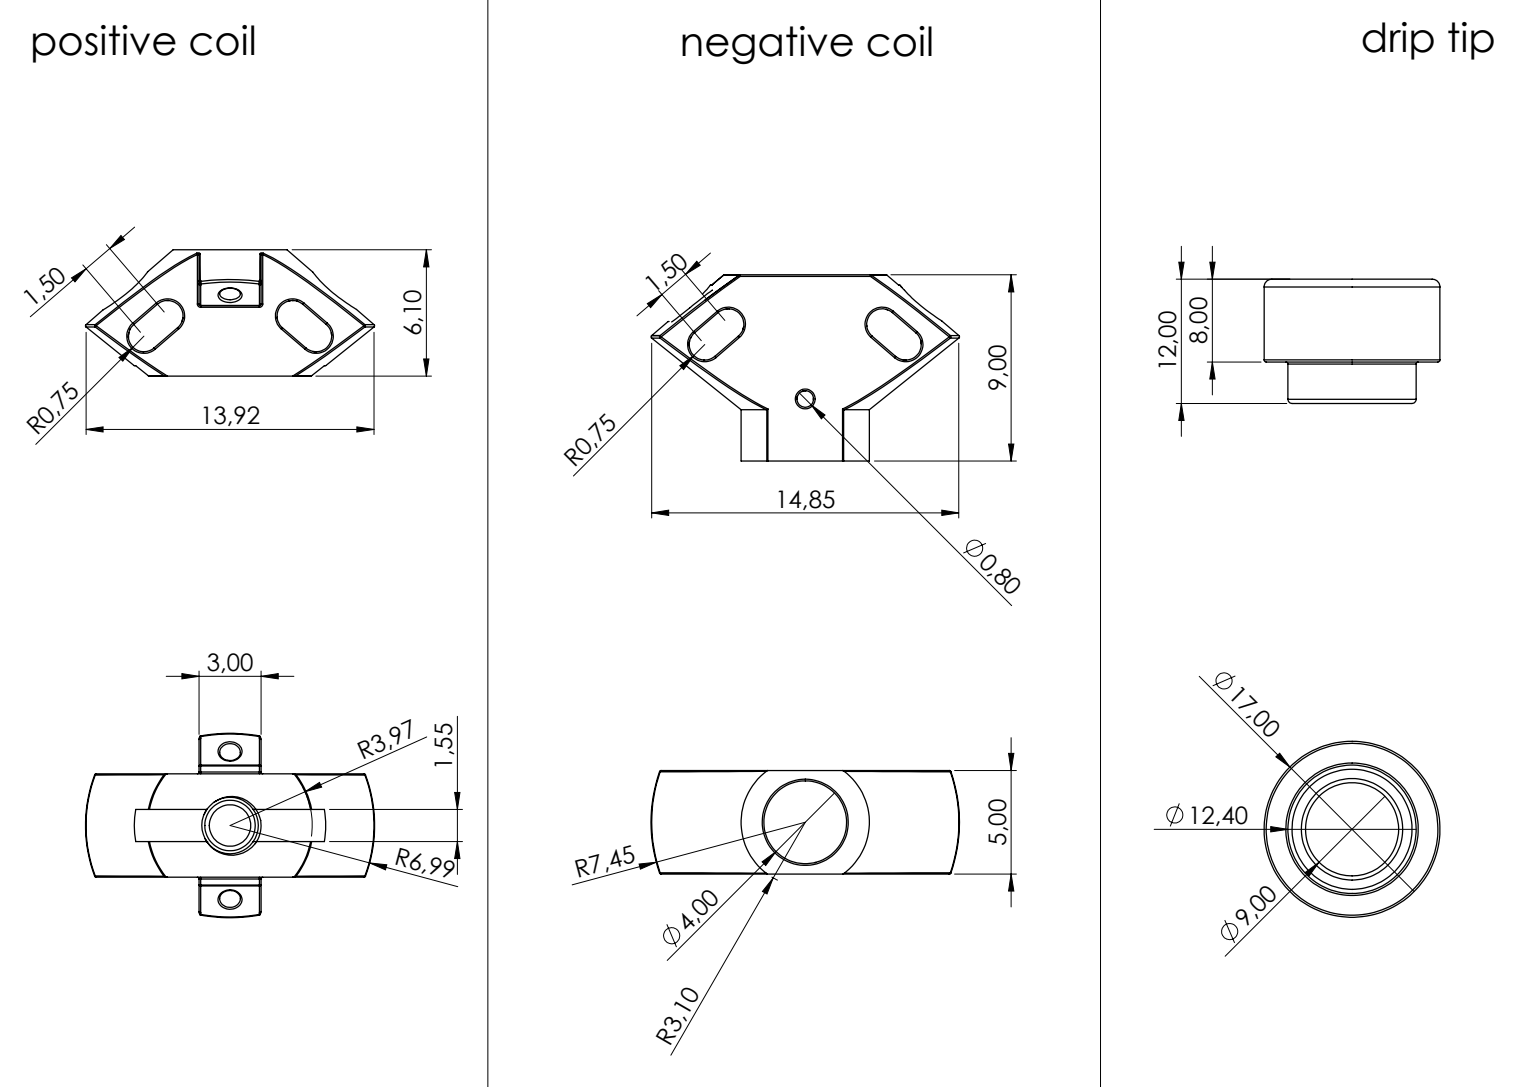
ISO-10303-21;
HEADER;
FILE_DESCRIPTION (('STEP AP214'),
    '1' );
FILE_NAME ('drip tip.step',
    '2026-10-05T20:10:51',
    ( '' ),
    ( '' ),
    'SwSTEP 2.0',
    'SolidWorks 2020',
    '' );
FILE_SCHEMA (( 'AUTOMOTIVE_DESIGN' ));
ENDSEC;

DATA;
#264=CARTESIAN_POINT ( 'NONE',  ( 0.000000000000000000, 6.999999999999992006, 4.500000000000000000 ) ) ;
#345=( NAMED_UNIT ( * ) PLANE_ANGLE_UNIT ( ) SI_UNIT ( $, .RADIAN. ) );
#574=EDGE_CURVE ( 'NONE', #72143, #200201, #108968, .T. ) ;
#1305=CARTESIAN_POINT ( 'NONE',  ( 0.000000000000000000, 10.00000000000000888, 0.000000000000000000 ) ) ;
#1373=EDGE_CURVE ( 'NONE', #149611, #126977, #18598, .T. ) ;
#1519=CARTESIAN_POINT ( 'NONE',  ( 0.000000000000000000, 6.999999999999992006, 0.000000000000000000 ) ) ;
#2109=VERTEX_POINT ( 'NONE', #48401 ) ;
#2320=CARTESIAN_POINT ( 'NONE',  ( 0.000000000000000000, -3.600000000000005862, 0.000000000000000000 ) ) ;
#2591=EDGE_CURVE ( 'NONE', #127623, #140029, #92727, .T. ) ;
#3387=DIRECTION ( 'NONE',  ( 0.000000000000000000, 0.000000000000000000, 1.000000000000000000 ) ) ;
#3603=ADVANCED_FACE ( 'NONE', ( #77901 ), #61609, .T. ) ;
#3770=ADVANCED_FACE ( 'NONE', ( #43300, #210018 ), #44358, .F. ) ;
#3987=CARTESIAN_POINT ( 'NONE',  ( 0.000000000000000000, 6.999999999999992006, 0.000000000000000000 ) ) ;
#4305=FACE_BOUND ( 'NONE', #212026, .T. ) ;
#4938=DIRECTION ( 'NONE',  ( 0.000000000000000000, 0.000000000000000000, 1.000000000000000000 ) ) ;
#5232=DIRECTION ( 'NONE',  ( 0.000000000000000000, -1.000000000000000000, 0.000000000000000000 ) ) ;
#5776=AXIS2_PLACEMENT_3D ( 'NONE', #186216, #103926, #18384 ) ;
#5884=( GEOMETRIC_REPRESENTATION_CONTEXT ( 3 ) GLOBAL_UNCERTAINTY_ASSIGNED_CONTEXT ( ( #116588 ) ) GLOBAL_UNIT_ASSIGNED_CONTEXT ( ( #15813, #115528, #82956 ) ) REPRESENTATION_CONTEXT ( 'NONE', 'WORKASPACE' ) );
#6450=CARTESIAN_POINT ( 'NONE',  ( 7.837739514543059934E-16, -0.2000000000000057288, -6.399999999999999467 ) ) ;
#7360=AXIS2_PLACEMENT_3D ( 'NONE', #71860, #19921, #90286 ) ;
#7540=ADVANCED_FACE ( 'NONE', ( #18411 ), #133280, .F. ) ;
#7671=CARTESIAN_POINT ( 'NONE',  ( 0.000000000000000000, 6.999999999999992006, 0.000000000000000000 ) ) ;
#7758=VECTOR ( 'NONE', #72110, 1000.000000000000000 ) ;
#8001=VECTOR ( 'NONE', #60877, 1000.000000000000000 ) ;
#8061=CIRCLE ( 'NONE', #129250, 7.750000000000000888 ) ;
#8134=VERTEX_POINT ( 'NONE', #207931 ) ;
#8319=CARTESIAN_POINT ( 'NONE',  ( 0.000000000000000000, -2.859583229930517945E-15, 6.399999999999999467 ) ) ;
#8641=AXIS2_PLACEMENT_3D ( 'NONE', #31169, #131895, #29033 ) ;
#9557=EDGE_LOOP ( 'NONE', ( #101500, #18562 ) ) ;
#9612=DIRECTION ( 'NONE',  ( 0.000000000000000000, 0.000000000000000000, 1.000000000000000000 ) ) ;
#9696=DIRECTION ( 'NONE',  ( 0.000000000000000000, 0.000000000000000000, 1.000000000000000000 ) ) ;
#9815=FACE_OUTER_BOUND ( 'NONE', #133822, .T. ) ;
#9854=DIRECTION ( 'NONE',  ( 0.000000000000000000, 0.000000000000000000, -1.000000000000000000 ) ) ;
#10274=EDGE_CURVE ( 'NONE', #26370, #93781, #171269, .T. ) ;
#10560=ORIENTED_EDGE ( 'NONE', *, *, #10274, .F. ) ;
#10650=ORIENTED_EDGE ( 'NONE', *, *, #170575, .T. ) ;
#10651=AXIS2_PLACEMENT_3D ( 'NONE', #60312, #126471, #44089 ) ;
#11410=EDGE_CURVE ( 'NONE', #127623, #2109, #69198, .T. ) ;
#11539=CIRCLE ( 'NONE', #136023, 0.4000000000000001887 ) ;
#11722=DIRECTION ( 'NONE',  ( 0.000000000000000000, -1.000000000000000000, 0.000000000000000000 ) ) ;
#12006=EDGE_CURVE ( 'NONE', #164855, #93781, #55325, .T. ) ;
#13222=CYLINDRICAL_SURFACE ( 'NONE', #176127, 8.500000000000000000 ) ;
#13360=DIRECTION ( 'NONE',  ( 0.000000000000000000, 0.000000000000000000, -1.000000000000000000 ) ) ;
#13864=DIRECTION ( 'NONE',  ( 0.000000000000000000, 0.000000000000000000, 1.000000000000000000 ) ) ;
#14011=CARTESIAN_POINT ( 'NONE',  ( 0.000000000000000000, 7.999999999999992895, 0.000000000000000000 ) ) ;
#14188=CIRCLE ( 'NONE', #135302, 0.4000000000000001887 ) ;
#14192=DIRECTION ( 'NONE',  ( 1.000000000000000000, -0.000000000000000000, 1.224646799147353207E-16 ) ) ;
#14250=CARTESIAN_POINT ( 'NONE',  ( 0.000000000000000000, -4.000000000000003553, 0.000000000000000000 ) ) ;
#15020=CARTESIAN_POINT ( 'NONE',  ( 1.028703311283776586E-15, 0.000000000000000000, -8.300000000000000711 ) ) ;
#15073=EDGE_CURVE ( 'NONE', #23490, #200201, #150501, .T. ) ;
#15171=AXIS2_PLACEMENT_3D ( 'NONE', #14250, #80343, #32656 ) ;
#15196=DIRECTION ( 'NONE',  ( 0.000000000000000000, 0.000000000000000000, 1.000000000000000000 ) ) ;
#15813=( LENGTH_UNIT ( ) NAMED_UNIT ( * ) SI_UNIT ( .MILLI., .METRE. ) );
#16136=AXIS2_PLACEMENT_3D ( 'NONE', #83388, #118101, #149472 ) ;
#16497=CARTESIAN_POINT ( 'NONE',  ( 7.592810154713589835E-16, -0.2000000000000057288, -6.200000000000000178 ) ) ;
#16828=EDGE_CURVE ( 'NONE', #71815, #212637, #195967, .T. ) ;
#16875=PRESENTATION_STYLE_ASSIGNMENT (( #180474 ) ) ;
#16964=ORIENTED_EDGE ( 'NONE', *, *, #574, .T. ) ;
#17327=EDGE_LOOP ( 'NONE', ( #66567, #70195, #176527, #91238 ) ) ;
#17374=DIRECTION ( 'NONE',  ( 0.000000000000000000, 0.000000000000000000, 1.000000000000000000 ) ) ;
#17603=AXIS2_PLACEMENT_3D ( 'NONE', #196348, #163856, #51161 ) ;
#17738=AXIS2_PLACEMENT_3D ( 'NONE', #106614, #187797, #189939 ) ;
#18384=DIRECTION ( 'NONE',  ( 0.000000000000000000, 0.000000000000000000, -1.000000000000000000 ) ) ;
#18411=FACE_OUTER_BOUND ( 'NONE', #115151, .T. ) ;
#18447=DIRECTION ( 'NONE',  ( 0.000000000000000000, 1.000000000000000000, 0.000000000000000000 ) ) ;
#18562=ORIENTED_EDGE ( 'NONE', *, *, #16828, .T. ) ;
#18598=CIRCLE ( 'NONE', #188047, 8.500000000000000000 ) ;
#18751=( NAMED_UNIT ( * ) SI_UNIT ( $, .STERADIAN. ) SOLID_ANGLE_UNIT ( ) );
#18967=AXIS2_PLACEMENT_3D ( 'NONE', #44218, #41025, #107134 ) ;
#19216=MANIFOLD_SOLID_BREP ( 'Fillet3', #122762 ) ;
#19595=ORIENTED_EDGE ( 'NONE', *, *, #112110, .T. ) ;
#19921=DIRECTION ( 'NONE',  ( 0.000000000000000000, 1.000000000000000000, 0.000000000000000000 ) ) ;
#19971=CARTESIAN_POINT ( 'NONE',  ( 0.000000000000000000, 7.999999999999992895, 0.000000000000000000 ) ) ;
#20632=DIRECTION ( 'NONE',  ( 0.000000000000000000, 1.000000000000000000, 0.000000000000000000 ) ) ;
#20648=VERTEX_POINT ( 'NONE', #121412 ) ;
#21650=DIRECTION ( 'NONE',  ( 0.000000000000000000, 0.000000000000000000, 1.000000000000000000 ) ) ;
#22091=ORIENTED_EDGE ( 'NONE', *, *, #182300, .F. ) ;
#22316=ORIENTED_EDGE ( 'NONE', *, *, #129911, .F. ) ;
#22969=CARTESIAN_POINT ( 'NONE',  ( 1.040949779275250140E-15, 7.250000000000006217, 8.500000000000000000 ) ) ;
#23415=EDGE_CURVE ( 'NONE', #172991, #155330, #176228, .T. ) ;
#23490=VERTEX_POINT ( 'NONE', #203951 ) ;
#23563=DIRECTION ( 'NONE',  ( 0.000000000000000000, 1.000000000000000000, 0.000000000000000000 ) ) ;
#24294=( GEOMETRIC_REPRESENTATION_CONTEXT ( 3 ) GLOBAL_UNCERTAINTY_ASSIGNED_CONTEXT ( ( #165204 ) ) GLOBAL_UNIT_ASSIGNED_CONTEXT ( ( #49154, #167164, #18751 ) ) REPRESENTATION_CONTEXT ( 'NONE', 'WORKASPACE' ) );
#24424=EDGE_CURVE ( 'NONE', #186457, #26370, #72606, .T. ) ;
#25000=AXIS2_PLACEMENT_3D ( 'NONE', #1305, #30653, #194198 ) ;
#25013=CARTESIAN_POINT ( 'NONE',  ( 0.000000000000000000, -4.000000000000003553, 6.200000000000000178 ) ) ;
#25180=CIRCLE ( 'NONE', #153201, 4.500000000000000000 ) ;
#25539=AXIS2_PLACEMENT_3D ( 'NONE', #92231, #106371, #172394 ) ;
#25943=FACE_OUTER_BOUND ( 'NONE', #203281, .T. ) ;
#26067=AXIS2_PLACEMENT_3D ( 'NONE', #122402, #89831, #9612 ) ;
#26099=ORIENTED_EDGE ( 'NONE', *, *, #129911, .T. ) ;
#26104=EDGE_LOOP ( 'NONE', ( #106132, #155824 ) ) ;
#26370=VERTEX_POINT ( 'NONE', #72434 ) ;
#27243=EDGE_LOOP ( 'NONE', ( #151851, #145363, #68319, #56562 ) ) ;
#27318=ORIENTED_EDGE ( 'NONE', *, *, #175406, .F. ) ;
#28088=ADVANCED_FACE ( 'NONE', ( #103376 ), #151075, .T. ) ;
#28593=VECTOR ( 'NONE', #183309, 1000.000000000000114 ) ;
#28786=ORIENTED_EDGE ( 'NONE', *, *, #197101, .F. ) ;
#29033=DIRECTION ( 'NONE',  ( 0.000000000000000000, 0.000000000000000000, 1.000000000000000000 ) ) ;
#29391=DIRECTION ( 'NONE',  ( 0.000000000000000000, 0.000000000000000000, -1.000000000000000000 ) ) ;
#29487=FACE_OUTER_BOUND ( 'NONE', #59958, .T. ) ;
#29491=ORIENTED_EDGE ( 'NONE', *, *, #2591, .F. ) ;
#29764=EDGE_LOOP ( 'NONE', ( #129103, #156266, #53842, #117131 ) ) ;
#30232=DIRECTION ( 'NONE',  ( 0.000000000000000000, 1.000000000000000000, 0.000000000000000000 ) ) ;
#30647=DIRECTION ( 'NONE',  ( 0.000000000000000000, 1.000000000000000000, 0.000000000000000000 ) ) ;
#30653=DIRECTION ( 'NONE',  ( 0.000000000000000000, -1.000000000000000000, 0.000000000000000000 ) ) ;
#30738=CARTESIAN_POINT ( 'NONE',  ( 0.000000000000000000, -4.000000000000005329, -4.899999999999999467 ) ) ;
#31169=CARTESIAN_POINT ( 'NONE',  ( 0.000000000000000000, 6.999999999999992006, 0.000000000000000000 ) ) ;
#31690=PRODUCT ( 'drip tip', 'drip tip', '', ( #82954 ) ) ;
#31977=CARTESIAN_POINT ( 'NONE',  ( 7.102951435054647665E-16, -3.600000000000005862, 5.799999999999999822 ) ) ;
#32090=EDGE_CURVE ( 'NONE', #20648, #185214, #46033, .T. ) ;
#32238=AXIS2_PLACEMENT_3D ( 'NONE', #93763, #127396, #73202 ) ;
#32423=DIRECTION ( 'NONE',  ( 0.000000000000000000, 0.000000000000000000, 1.000000000000000000 ) ) ;
#32656=DIRECTION ( 'NONE',  ( 0.000000000000000000, 0.000000000000000000, -1.000000000000000000 ) ) ;
#32807=DIRECTION ( 'NONE',  ( 0.000000000000000000, 0.000000000000000000, -1.000000000000000000 ) ) ;
#33263=EDGE_LOOP ( 'NONE', ( #160788, #202164 ) ) ;
#33961=DIRECTION ( 'NONE',  ( 0.000000000000000000, -1.000000000000000000, 0.000000000000000000 ) ) ;
#34059=DIRECTION ( 'NONE',  ( 0.000000000000000000, -1.000000000000000000, 0.000000000000000000 ) ) ;
#34206=SURFACE_STYLE_FILL_AREA ( #64591 ) ;
#34411=AXIS2_PLACEMENT_3D ( 'NONE', #199703, #200761, #52411 ) ;
#34430=VECTOR ( 'NONE', #188585, 1000.000000000000000 ) ;
#34590=DIRECTION ( 'NONE',  ( 8.659560562354940254E-17, 0.7071067811865469066, -0.7071067811865481278 ) ) ;
#36222=DIRECTION ( 'NONE',  ( 0.000000000000000000, -1.000000000000000000, 0.000000000000000000 ) ) ;
#36564=DIRECTION ( 'NONE',  ( 1.000000000000000000, 0.000000000000000000, -1.224646799147353207E-16 ) ) ;
#36794=DIRECTION ( 'NONE',  ( 0.000000000000000000, -1.000000000000000000, 0.000000000000000000 ) ) ;
#36987=ORIENTED_EDGE ( 'NONE', *, *, #40952, .T. ) ;
#37772=CARTESIAN_POINT ( 'NONE',  ( 0.000000000000000000, 10.00000000000000888, -4.500000000000000000 ) ) ;
#38119=CARTESIAN_POINT ( 'NONE',  ( 7.592810154713589835E-16, -3.600000000000005862, -6.200000000000000178 ) ) ;
#38330=CARTESIAN_POINT ( 'NONE',  ( 0.000000000000000000, -3.600000000000005862, 0.000000000000000000 ) ) ;
#39003=CIRCLE ( 'NONE', #70207, 0.1999999999999996503 ) ;
#39310=ORIENTED_EDGE ( 'NONE', *, *, #12006, .F. ) ;
#39390=FACE_OUTER_BOUND ( 'NONE', #145990, .T. ) ;
#39682=CIRCLE ( 'NONE', #74325, 8.500000000000000000 ) ;
#39879=CARTESIAN_POINT ( 'NONE',  ( 7.837739514543059934E-16, -2.859583229930517945E-15, -6.399999999999999467 ) ) ;
#40809=TOROIDAL_SURFACE ( 'NONE', #193078, 4.899999999999999467, 0.4000000000000000222 ) ;
#40952=EDGE_CURVE ( 'NONE', #93781, #164855, #200207, .T. ) ;
#41025=DIRECTION ( 'NONE',  ( -0.000000000000000000, 1.000000000000000000, -0.000000000000000000 ) ) ;
#41110=DIRECTION ( 'NONE',  ( -1.000000000000000000, -0.000000000000000000, -0.000000000000000000 ) ) ;
#41149=AXIS2_PLACEMENT_3D ( 'NONE', #200524, #52170, #3387 ) ;
#41923=DIRECTION ( 'NONE',  ( 0.000000000000000000, 0.000000000000000000, 1.000000000000000000 ) ) ;
#42907=ADVANCED_FACE ( 'NONE', ( #29487 ), #13222, .T. ) ;
#42957=TOROIDAL_SURFACE ( 'NONE', #63644, 8.300000000000000711, 0.2000000000000000111 ) ;
#43300=FACE_BOUND ( 'NONE', #9557, .T. ) ;
#43703=DIRECTION ( 'NONE',  ( 0.000000000000000000, 0.000000000000000000, 1.000000000000000000 ) ) ;
#44089=DIRECTION ( 'NONE',  ( 0.000000000000000000, 0.000000000000000000, 1.000000000000000000 ) ) ;
#44218=CARTESIAN_POINT ( 'NONE',  ( 0.000000000000000000, -4.000000000000003553, 0.000000000000000000 ) ) ;
#44358=PLANE ( 'NONE',  #151465 ) ;
#44912=ORIENTED_EDGE ( 'NONE', *, *, #191183, .F. ) ;
#45289=DIRECTION ( 'NONE',  ( 1.224646799147353454E-16, 0.000000000000000000, -1.000000000000000000 ) ) ;
#45646=ORIENTED_EDGE ( 'NONE', *, *, #24424, .F. ) ;
#45992=AXIS2_PLACEMENT_3D ( 'NONE', #166851, #18447, #136493 ) ;
#45996=AXIS2_PLACEMENT_3D ( 'NONE', #1519, #82797, #197608 ) ;
#46033=CIRCLE ( 'NONE', #32238, 4.500000000000000000 ) ;
#46107=DIRECTION ( 'NONE',  ( 1.000000000000000000, 0.000000000000000000, -1.224646799147353207E-16 ) ) ;
#46353=DIRECTION ( 'NONE',  ( 1.000000000000000000, -0.000000000000000000, 1.224646799147353207E-16 ) ) ;
#46679=ORIENTED_EDGE ( 'NONE', *, *, #40952, .F. ) ;
#47576=AXIS2_PLACEMENT_3D ( 'NONE', #3987, #182755, #200066 ) ;
#48401=CARTESIAN_POINT ( 'NONE',  ( 9.950255243072246565E-16, 7.999999999999992895, -7.750000000000000888 ) ) ;
#48862=CARTESIAN_POINT ( 'NONE',  ( 1.016456843292303031E-15, 0.2000000000000057288, -8.300000000000000711 ) ) ;
#49154=( LENGTH_UNIT ( ) NAMED_UNIT ( * ) SI_UNIT ( .MILLI., .METRE. ) );
#50211=( NAMED_UNIT ( * ) SI_UNIT ( $, .STERADIAN. ) SOLID_ANGLE_UNIT ( ) );
#51161=DIRECTION ( 'NONE',  ( 0.000000000000000000, 0.000000000000000000, 1.000000000000000000 ) ) ;
#51278=DIRECTION ( 'NONE',  ( -1.000000000000000000, 0.000000000000000000, 0.000000000000000000 ) ) ;
#52170=DIRECTION ( 'NONE',  ( -0.000000000000000000, -1.000000000000000000, -0.000000000000000000 ) ) ;
#52411=DIRECTION ( 'NONE',  ( 0.000000000000000000, 0.000000000000000000, -1.000000000000000000 ) ) ;
#52834=ADVANCED_FACE ( 'NONE', ( #132656 ), #177396, .F. ) ;
#53318=LINE ( 'NONE', #264, #28593 ) ;
#53399=FILL_AREA_STYLE_COLOUR ( '', #190373 ) ;
#53512=DIRECTION ( 'NONE',  ( 0.000000000000000000, 0.000000000000000000, -1.000000000000000000 ) ) ;
#53589=CIRCLE ( 'NONE', #188407, 8.500000000000000000 ) ;
#53842=ORIENTED_EDGE ( 'NONE', *, *, #175406, .T. ) ;
#55192=ADVANCED_BREP_SHAPE_REPRESENTATION ( '', ( #19216, #200407 ), #152191 ) ;
#55325=CIRCLE ( 'NONE', #131441, 6.200000000000000178 ) ;
#55431=FACE_OUTER_BOUND ( 'NONE', #211433, .T. ) ;
#55551=EDGE_CURVE ( 'NONE', #132973, #2109, #8061, .T. ) ;
#56102=CARTESIAN_POINT ( 'NONE',  ( 0.000000000000000000, 0.000000000000000000, 0.000000000000000000 ) ) ;
#56254=ORIENTED_EDGE ( 'NONE', *, *, #80870, .F. ) ;
#56298=DIRECTION ( 'NONE',  ( 1.224646799147353454E-16, 0.000000000000000000, -1.000000000000000000 ) ) ;
#56425=AXIS2_PLACEMENT_3D ( 'NONE', #78190, #94472, #162661 ) ;
#56562=ORIENTED_EDGE ( 'NONE', *, *, #57451, .F. ) ;
#56611=DIRECTION ( 'NONE',  ( -1.000000000000000000, -0.000000000000000000, -0.000000000000000000 ) ) ;
#57451=EDGE_CURVE ( 'NONE', #23490, #185214, #106026, .T. ) ;
#57610=CONICAL_SURFACE ( 'NONE', #199358, 4.500000000000000000, 0.7853981633974491672 ) ;
#58396=ORIENTED_EDGE ( 'NONE', *, *, #55551, .F. ) ;
#59841=DIRECTION ( 'NONE',  ( 0.000000000000000000, 0.000000000000000000, -1.000000000000000000 ) ) ;
#59958=EDGE_LOOP ( 'NONE', ( #175177, #175570, #88728, #105076 ) ) ;
#60312=CARTESIAN_POINT ( 'NONE',  ( 0.000000000000000000, 0.2000000000000057288, 8.300000000000000711 ) ) ;
#60877=DIRECTION ( 'NONE',  ( 0.000000000000000000, -1.000000000000000000, 0.000000000000000000 ) ) ;
#61609=TOROIDAL_SURFACE ( 'NONE', #134169, 7.750000000000000888, 0.7500000000000000000 ) ;
#62655=VECTOR ( 'NONE', #5232, 1000.000000000000000 ) ;
#62703=EDGE_LOOP ( 'NONE', ( #56254, #70105, #185472, #36987 ) ) ;
#63508=CIRCLE ( 'NONE', #87776, 0.4000000000000001887 ) ;
#63620=EDGE_CURVE ( 'NONE', #163746, #20648, #205318, .T. ) ;
#63644=AXIS2_PLACEMENT_3D ( 'NONE', #188449, #92050, #9696 ) ;
#64591=FILL_AREA_STYLE ('',( #98177 ) ) ;
#65210=ADVANCED_FACE ( 'NONE', ( #185205, #4305 ), #200386, .T. ) ;
#65319=EDGE_CURVE ( 'NONE', #71815, #164855, #39003, .T. ) ;
#65544=UNCERTAINTY_MEASURE_WITH_UNIT (LENGTH_MEASURE( 1.000000000000000082E-05 ), #116330, 'distance_accuracy_value', 'NONE');
#66252=FACE_OUTER_BOUND ( 'NONE', #17327, .T. ) ;
#66418=SURFACE_STYLE_FILL_AREA ( #199633 ) ;
#66567=ORIENTED_EDGE ( 'NONE', *, *, #112110, .F. ) ;
#67883=ORIENTED_EDGE ( 'NONE', *, *, #12006, .T. ) ;
#68319=ORIENTED_EDGE ( 'NONE', *, *, #32090, .T. ) ;
#68577=ADVANCED_FACE ( 'NONE', ( #135841 ), #181091, .T. ) ;
#69198=CIRCLE ( 'NONE', #103721, 0.7499999999999997780 ) ;
#69352=CARTESIAN_POINT ( 'NONE',  ( 0.000000000000000000, 7.250000000000006217, -8.500000000000000000 ) ) ;
#69541=CARTESIAN_POINT ( 'NONE',  ( 0.000000000000000000, -3.600000000000005862, 0.000000000000000000 ) ) ;
#69625=ADVANCED_FACE ( 'NONE', ( #55431 ), #174308, .T. ) ;
#69627=SHAPE_REPRESENTATION_RELATIONSHIP ( 'NONE' , 'NONE' ,  #188305, #55192 ) ;
#69891=ADVANCED_FACE ( 'NONE', ( #96624, #127054 ), #178931, .T. ) ;
#70105=ORIENTED_EDGE ( 'NONE', *, *, #24424, .T. ) ;
#70195=ORIENTED_EDGE ( 'NONE', *, *, #162297, .F. ) ;
#70207=AXIS2_PLACEMENT_3D ( 'NONE', #6450, #175392, #56298 ) ;
#70299=CIRCLE ( 'NONE', #56425, 8.300000000000000711 ) ;
#70727=TOROIDAL_SURFACE ( 'NONE', #191810, 4.899999999999999467, 0.4000000000000000222 ) ;
#71617=STYLED_ITEM ( 'NONE', ( #16875 ), #19216 ) ;
#71769=ORIENTED_EDGE ( 'NONE', *, *, #57451, .T. ) ;
#71815=VERTEX_POINT ( 'NONE', #39879 ) ;
#71860=CARTESIAN_POINT ( 'NONE',  ( 0.000000000000000000, 7.250000000000006217, 0.000000000000000000 ) ) ;
#72110=DIRECTION ( 'NONE',  ( 0.000000000000000000, -1.000000000000000000, 0.000000000000000000 ) ) ;
#72143=VERTEX_POINT ( 'NONE', #91850 ) ;
#72434=CARTESIAN_POINT ( 'NONE',  ( 0.000000000000000000, -3.600000000000005862, 6.200000000000000178 ) ) ;
#72606=CIRCLE ( 'NONE', #34411, 6.200000000000000178 ) ;
#72771=ADVANCED_FACE ( 'NONE', ( #123894 ), #194160, .F. ) ;
#72991=ORIENTED_EDGE ( 'NONE', *, *, #170575, .F. ) ;
#73202=DIRECTION ( 'NONE',  ( 0.000000000000000000, 0.000000000000000000, -1.000000000000000000 ) ) ;
#73702=VECTOR ( 'NONE', #23563, 1000.000000000000000 ) ;
#74162=ADVANCED_FACE ( 'NONE', ( #39390 ), #166470, .T. ) ;
#74325=AXIS2_PLACEMENT_3D ( 'NONE', #98338, #182770, #13864 ) ;
#75338=CARTESIAN_POINT ( 'NONE',  ( 5.510910596163088569E-16, 10.00000000000000888, 4.500000000000000000 ) ) ;
#76218=CARTESIAN_POINT ( 'NONE',  ( 7.347880794884118750E-16, -4.000000000000003553, 5.799999999999999822 ) ) ;
#77901=FACE_OUTER_BOUND ( 'NONE', #29764, .T. ) ;
#78190=CARTESIAN_POINT ( 'NONE',  ( 0.000000000000000000, 0.000000000000000000, 0.000000000000000000 ) ) ;
#78964=DIRECTION ( 'NONE',  ( 0.000000000000000000, 0.000000000000000000, 1.000000000000000000 ) ) ;
#79154=EDGE_LOOP ( 'NONE', ( #209645, #149612, #67883, #10560 ) ) ;
#79158=ORIENTED_EDGE ( 'NONE', *, *, #87756, .F. ) ;
#79202=ORIENTED_EDGE ( 'NONE', *, *, #163561, .F. ) ;
#79679=STYLED_ITEM ( 'NONE', ( #151982 ), #55192 ) ;
#80179=ORIENTED_EDGE ( 'NONE', *, *, #179626, .T. ) ;
#80292=VERTEX_POINT ( 'NONE', #15020 ) ;
#80343=DIRECTION ( 'NONE',  ( 0.000000000000000000, -1.000000000000000000, 0.000000000000000000 ) ) ;
#80524=CIRCLE ( 'NONE', #198166, 5.500000000000005329 ) ;
#80870=EDGE_CURVE ( 'NONE', #186457, #164855, #190333, .T. ) ;
#81525=FACE_OUTER_BOUND ( 'NONE', #79154, .T. ) ;
#82404=CARTESIAN_POINT ( 'NONE',  ( 0.000000000000000000, 0.000000000000000000, 8.300000000000000711 ) ) ;
#82529=DIRECTION ( 'NONE',  ( 0.000000000000000000, -1.000000000000000000, 0.000000000000000000 ) ) ;
#82575=FACE_OUTER_BOUND ( 'NONE', #27243, .T. ) ;
#82609=DIRECTION ( 'NONE',  ( 0.000000000000000000, -1.000000000000000000, 0.000000000000000000 ) ) ;
#82797=DIRECTION ( 'NONE',  ( 0.000000000000000000, 1.000000000000000000, 0.000000000000000000 ) ) ;
#82954=PRODUCT_CONTEXT ( 'NONE', #201209, 'mechanical' ) ;
#82956=( NAMED_UNIT ( * ) SI_UNIT ( $, .STERADIAN. ) SOLID_ANGLE_UNIT ( ) );
#83331=CARTESIAN_POINT ( 'NONE',  ( 5.510910596163088569E-16, 6.999999999999992006, -4.500000000000000000 ) ) ;
#83388=CARTESIAN_POINT ( 'NONE',  ( 0.000000000000000000, 0.000000000000000000, 0.000000000000000000 ) ) ;
#83645=EDGE_LOOP ( 'NONE', ( #177931, #80179 ) ) ;
#83982=VERTEX_POINT ( 'NONE', #30738 ) ;
#86161=SHAPE_DEFINITION_REPRESENTATION ( #128549, #188305 ) ;
#86301=CARTESIAN_POINT ( 'NONE',  ( 6.735557395310444981E-16, 7.999999999999992895, -5.500000000000002665 ) ) ;
#86971=CARTESIAN_POINT ( 'NONE',  ( 0.000000000000000000, -0.2000000000000057288, 6.399999999999999467 ) ) ;
#87756=EDGE_CURVE ( 'NONE', #23490, #163746, #150598, .T. ) ;
#87776=AXIS2_PLACEMENT_3D ( 'NONE', #108622, #56611, #122775 ) ;
#88728=ORIENTED_EDGE ( 'NONE', *, *, #192353, .T. ) ;
#89166=CIRCLE ( 'NONE', #47576, 4.500000000000000000 ) ;
#89189=DIRECTION ( 'NONE',  ( 0.000000000000000000, -1.000000000000000000, 0.000000000000000000 ) ) ;
#89831=DIRECTION ( 'NONE',  ( 0.000000000000000000, 1.000000000000000000, 0.000000000000000000 ) ) ;
#90286=DIRECTION ( 'NONE',  ( 0.000000000000000000, 0.000000000000000000, 1.000000000000000000 ) ) ;
#91238=ORIENTED_EDGE ( 'NONE', *, *, #32090, .F. ) ;
#91398=EDGE_CURVE ( 'NONE', #8134, #83982, #174578, .T. ) ;
#91569=CIRCLE ( 'NONE', #119276, 0.4000000000000001887 ) ;
#91812=CARTESIAN_POINT ( 'NONE',  ( 7.592810154713589835E-16, -4.000000000000003553, -6.200000000000000178 ) ) ;
#91850=CARTESIAN_POINT ( 'NONE',  ( 0.000000000000000000, 7.999999999999992895, 5.500000000000002665 ) ) ;
#92050=DIRECTION ( 'NONE',  ( 0.000000000000000000, 1.000000000000000000, 0.000000000000000000 ) ) ;
#92213=CARTESIAN_POINT ( 'NONE',  ( 0.000000000000000000, -3.600000000000005862, 0.000000000000000000 ) ) ;
#92231=CARTESIAN_POINT ( 'NONE',  ( 0.000000000000000000, 0.2000000000000057288, 0.000000000000000000 ) ) ;
#92573=AXIS2_PLACEMENT_3D ( 'NONE', #160121, #11722, #144972 ) ;
#92593=CARTESIAN_POINT ( 'NONE',  ( 0.000000000000000000, -0.2000000000000057288, 0.000000000000000000 ) ) ;
#92727=CIRCLE ( 'NONE', #123875, 8.500000000000000000 ) ;
#93763=CARTESIAN_POINT ( 'NONE',  ( 0.000000000000000000, -3.600000000000005862, 0.000000000000000000 ) ) ;
#93781=VERTEX_POINT ( 'NONE', #162520 ) ;
#94472=DIRECTION ( 'NONE',  ( -0.000000000000000000, -1.000000000000000000, -0.000000000000000000 ) ) ;
#94856=DIRECTION ( 'NONE',  ( -1.224646799147353207E-16, 0.000000000000000000, -1.000000000000000000 ) ) ;
#95216=CARTESIAN_POINT ( 'NONE',  ( 0.000000000000000000, 0.000000000000000000, 0.000000000000000000 ) ) ;
#96475=ORIENTED_EDGE ( 'NONE', *, *, #176945, .T. ) ;
#96624=FACE_OUTER_BOUND ( 'NONE', #26104, .T. ) ;
#97027=MECHANICAL_DESIGN_GEOMETRIC_PRESENTATION_REPRESENTATION('',(#79679),#24294);
#97143=CIRCLE ( 'NONE', #110934, 4.899999999999999467 ) ;
#97316=DIRECTION ( 'NONE',  ( 0.000000000000000000, 0.000000000000000000, 1.000000000000000000 ) ) ;
#97732=AXIS2_PLACEMENT_3D ( 'NONE', #205761, #186309, #21650 ) ;
#98177=FILL_AREA_STYLE_COLOUR ( '', #151279 ) ;
#98338=CARTESIAN_POINT ( 'NONE',  ( 0.000000000000000000, 7.250000000000006217, 0.000000000000000000 ) ) ;
#100037=LINE ( 'NONE', #169299, #119672 ) ;
#100775=CARTESIAN_POINT ( 'NONE',  ( 0.000000000000000000, 7.999999999999992895, 0.000000000000000000 ) ) ;
#101227=CIRCLE ( 'NONE', #194629, 0.2000000000000005107 ) ;
#101500=ORIENTED_EDGE ( 'NONE', *, *, #147855, .T. ) ;
#101870=ORIENTED_EDGE ( 'NONE', *, *, #179626, .F. ) ;
#101992=AXIS2_PLACEMENT_3D ( 'NONE', #162306, #193722, #97316 ) ;
#102157=SURFACE_SIDE_STYLE ('',( #66418 ) ) ;
#103141=ORIENTED_EDGE ( 'NONE', *, *, #15073, .F. ) ;
#103356=PRODUCT_DEFINITION ( 'UNKNOWN', '', #142178, #113337 ) ;
#103376=FACE_OUTER_BOUND ( 'NONE', #210209, .T. ) ;
#103721=AXIS2_PLACEMENT_3D ( 'NONE', #173170, #46353, #45289 ) ;
#103926=DIRECTION ( 'NONE',  ( 0.000000000000000000, -1.000000000000000000, 0.000000000000000000 ) ) ;
#103943=EDGE_LOOP ( 'NONE', ( #79158, #119377, #159598, #192403 ) ) ;
#105076=ORIENTED_EDGE ( 'NONE', *, *, #188776, .T. ) ;
#105980=ORIENTED_EDGE ( 'NONE', *, *, #130371, .F. ) ;
#106026=LINE ( 'NONE', #37772, #62655 ) ;
#106132=ORIENTED_EDGE ( 'NONE', *, *, #23415, .T. ) ;
#106371=DIRECTION ( 'NONE',  ( 0.000000000000000000, 1.000000000000000000, 0.000000000000000000 ) ) ;
#106614=CARTESIAN_POINT ( 'NONE',  ( 0.000000000000000000, -4.000000000000003553, 0.000000000000000000 ) ) ;
#107134=DIRECTION ( 'NONE',  ( 0.000000000000000000, 0.000000000000000000, -1.000000000000000000 ) ) ;
#108622=CARTESIAN_POINT ( 'NONE',  ( 0.000000000000000000, -3.600000000000005862, -5.799999999999999822 ) ) ;
#108881=DIRECTION ( 'NONE',  ( -0.000000000000000000, -1.000000000000000000, -0.000000000000000000 ) ) ;
#108968=CIRCLE ( 'NONE', #181551, 5.500000000000005329 ) ;
#109188=DIRECTION ( 'NONE',  ( 0.000000000000000000, 0.000000000000000000, 1.000000000000000000 ) ) ;
#109371=AXIS2_PLACEMENT_3D ( 'NONE', #149498, #36794, #152690 ) ;
#110009=ORIENTED_EDGE ( 'NONE', *, *, #65319, .T. ) ;
#110701=CARTESIAN_POINT ( 'NONE',  ( 0.000000000000000000, -3.600000000000005862, 0.000000000000000000 ) ) ;
#110934=AXIS2_PLACEMENT_3D ( 'NONE', #159621, #193179, #13360 ) ;
#111978=CIRCLE ( 'NONE', #125899, 0.1999999999999996503 ) ;
#112110=EDGE_CURVE ( 'NONE', #8134, #20648, #11539, .T. ) ;
#113337=PRODUCT_DEFINITION_CONTEXT ( 'detailed design', #169602, 'design' ) ;
#114279=EDGE_LOOP ( 'NONE', ( #44912, #10650, #195307, #22091 ) ) ;
#114475=SURFACE_SIDE_STYLE ('',( #34206 ) ) ;
#114745=AXIS2_PLACEMENT_3D ( 'NONE', #175767, #172561, #158440 ) ;
#115151=EDGE_LOOP ( 'NONE', ( #177846, #208584, #71769, #201906 ) ) ;
#115528=( NAMED_UNIT ( * ) PLANE_ANGLE_UNIT ( ) SI_UNIT ( $, .RADIAN. ) );
#115745=CARTESIAN_POINT ( 'NONE',  ( 6.000769315822030740E-16, -3.600000000000005862, 4.899999999999999467 ) ) ;
#116185=ADVANCED_FACE ( 'NONE', ( #25943 ), #42957, .T. ) ;
#116330=( LENGTH_UNIT ( ) NAMED_UNIT ( * ) SI_UNIT ( .MILLI., .METRE. ) );
#116588=UNCERTAINTY_MEASURE_WITH_UNIT (LENGTH_MEASURE( 1.000000000000000082E-05 ), #15813, 'distance_accuracy_value', 'NONE');
#117131=ORIENTED_EDGE ( 'NONE', *, *, #119697, .F. ) ;
#118101=DIRECTION ( 'NONE',  ( -0.000000000000000000, -1.000000000000000000, -0.000000000000000000 ) ) ;
#118618=DIRECTION ( 'NONE',  ( 0.000000000000000000, 0.000000000000000000, -1.000000000000000000 ) ) ;
#119276=AXIS2_PLACEMENT_3D ( 'NONE', #154845, #41110, #186254 ) ;
#119377=ORIENTED_EDGE ( 'NONE', *, *, #15073, .T. ) ;
#119672=VECTOR ( 'NONE', #33961, 1000.000000000000000 ) ;
#119697=EDGE_CURVE ( 'NONE', #2109, #132973, #171249, .T. ) ;
#119946=AXIS2_PLACEMENT_3D ( 'NONE', #192040, #30647, #43703 ) ;
#121412=CARTESIAN_POINT ( 'NONE',  ( 5.510910596163088569E-16, -3.600000000000005862, 4.500000000000000000 ) ) ;
#121754=CARTESIAN_POINT ( 'NONE',  ( 0.000000000000000000, -4.000000000000003553, 0.000000000000000000 ) ) ;
#122402=CARTESIAN_POINT ( 'NONE',  ( 0.000000000000000000, -0.2000000000000057288, 0.000000000000000000 ) ) ;
#122636=ORIENTED_EDGE ( 'NONE', *, *, #55551, .T. ) ;
#122762=CLOSED_SHELL ( 'NONE', ( #116185, #189849, #153001, #68577, #74162, #52834, #133317, #164766, #28088, #42907, #65210, #3770, #171652, #69891, #7540, #125806, #3603, #197146, #187447, #72771, #69625 ) ) ;
#122775=DIRECTION ( 'NONE',  ( 0.000000000000000000, 0.000000000000000000, 1.000000000000000000 ) ) ;
#123518=ORIENTED_EDGE ( 'NONE', *, *, #157520, .F. ) ;
#123608=EDGE_LOOP ( 'NONE', ( #72991, #45646, #143114, #138432 ) ) ;
#123875=AXIS2_PLACEMENT_3D ( 'NONE', #126430, #178313, #41923 ) ;
#123894=FACE_OUTER_BOUND ( 'NONE', #173536, .T. ) ;
#125470=CIRCLE ( 'NONE', #97732, 0.7499999999999997780 ) ;
#125806=ADVANCED_FACE ( 'NONE', ( #9815 ), #57610, .F. ) ;
#125899=AXIS2_PLACEMENT_3D ( 'NONE', #86971, #51278, #153041 ) ;
#126378=ORIENTED_EDGE ( 'NONE', *, *, #179502, .T. ) ;
#126430=CARTESIAN_POINT ( 'NONE',  ( 0.000000000000000000, 7.250000000000006217, 0.000000000000000000 ) ) ;
#126471=DIRECTION ( 'NONE',  ( -1.000000000000000000, 0.000000000000000000, 0.000000000000000000 ) ) ;
#126977=VERTEX_POINT ( 'NONE', #180269 ) ;
#127054=FACE_BOUND ( 'NONE', #33263, .T. ) ;
#127396=DIRECTION ( 'NONE',  ( 0.000000000000000000, -1.000000000000000000, 0.000000000000000000 ) ) ;
#127623=VERTEX_POINT ( 'NONE', #69352 ) ;
#127828=CARTESIAN_POINT ( 'NONE',  ( 0.000000000000000000, 0.000000000000000000, 0.000000000000000000 ) ) ;
#128549=PRODUCT_DEFINITION_SHAPE ( 'NONE', 'NONE',  #103356 ) ;
#128873=DIRECTION ( 'NONE',  ( 0.000000000000000000, 1.000000000000000000, 0.000000000000000000 ) ) ;
#129103=ORIENTED_EDGE ( 'NONE', *, *, #11410, .F. ) ;
#129250=AXIS2_PLACEMENT_3D ( 'NONE', #189062, #185842, #4938 ) ;
#129911=EDGE_CURVE ( 'NONE', #200201, #72143, #80524, .T. ) ;
#130319=VERTEX_POINT ( 'NONE', #82404 ) ;
#130356=CYLINDRICAL_SURFACE ( 'NONE', #17603, 6.200000000000000178 ) ;
#130371=EDGE_CURVE ( 'NONE', #80292, #126977, #101227, .T. ) ;
#130995=DIRECTION ( 'NONE',  ( 0.000000000000000000, 0.000000000000000000, 1.000000000000000000 ) ) ;
#131441=AXIS2_PLACEMENT_3D ( 'NONE', #92593, #108881, #191106 ) ;
#131803=ORIENTED_EDGE ( 'NONE', *, *, #163561, .T. ) ;
#131895=DIRECTION ( 'NONE',  ( 0.000000000000000000, 1.000000000000000000, 0.000000000000000000 ) ) ;
#132002=DIRECTION ( 'NONE',  ( 0.000000000000000000, 0.000000000000000000, 1.000000000000000000 ) ) ;
#132656=FACE_OUTER_BOUND ( 'NONE', #103943, .T. ) ;
#132778=ORIENTED_EDGE ( 'NONE', *, *, #91398, .F. ) ;
#132973=VERTEX_POINT ( 'NONE', #193130 ) ;
#133280=CYLINDRICAL_SURFACE ( 'NONE', #109371, 4.500000000000000000 ) ;
#133317=ADVANCED_FACE ( 'NONE', ( #82575 ), #163853, .F. ) ;
#133415=CIRCLE ( 'NONE', #164446, 6.200000000000000178 ) ;
#133822=EDGE_LOOP ( 'NONE', ( #103141, #180628, #96475, #22316 ) ) ;
#133861=TOROIDAL_SURFACE ( 'NONE', #5776, 5.799999999999999822, 0.4000000000000000222 ) ;
#134169=AXIS2_PLACEMENT_3D ( 'NONE', #178622, #128873, #130995 ) ;
#135162=CIRCLE ( 'NONE', #10651, 0.2000000000000005107 ) ;
#135172=ORIENTED_EDGE ( 'NONE', *, *, #147855, .F. ) ;
#135302=AXIS2_PLACEMENT_3D ( 'NONE', #31977, #46107, #94856 ) ;
#135841=FACE_OUTER_BOUND ( 'NONE', #114279, .T. ) ;
#136023=AXIS2_PLACEMENT_3D ( 'NONE', #115745, #36564, #150340 ) ;
#136493=DIRECTION ( 'NONE',  ( 0.000000000000000000, 0.000000000000000000, 1.000000000000000000 ) ) ;
#136499=DIRECTION ( 'NONE',  ( -0.000000000000000000, -1.000000000000000000, -0.000000000000000000 ) ) ;
#138432=ORIENTED_EDGE ( 'NONE', *, *, #200474, .F. ) ;
#139851=DIRECTION ( 'NONE',  ( 0.000000000000000000, 1.000000000000000000, 0.000000000000000000 ) ) ;
#140029=VERTEX_POINT ( 'NONE', #22969 ) ;
#140975=EDGE_LOOP ( 'NONE', ( #132778, #19595, #155052, #123518 ) ) ;
#141998=DIRECTION ( 'NONE',  ( 0.000000000000000000, 0.000000000000000000, 1.000000000000000000 ) ) ;
#142178=PRODUCT_DEFINITION_FORMATION_WITH_SPECIFIED_SOURCE ( 'ANY', '', #31690, .NOT_KNOWN. ) ;
#143114=ORIENTED_EDGE ( 'NONE', *, *, #182300, .T. ) ;
#144972=DIRECTION ( 'NONE',  ( 0.000000000000000000, 0.000000000000000000, -1.000000000000000000 ) ) ;
#145031=VECTOR ( 'NONE', #34590, 1000.000000000000114 ) ;
#145248=ORIENTED_EDGE ( 'NONE', *, *, #1373, .F. ) ;
#145363=ORIENTED_EDGE ( 'NONE', *, *, #63620, .T. ) ;
#145990=EDGE_LOOP ( 'NONE', ( #29491, #147733, #58396, #27318 ) ) ;
#147364=CARTESIAN_POINT ( 'NONE',  ( 0.000000000000000000, 0.2000000000000057288, 0.000000000000000000 ) ) ;
#147611=CIRCLE ( 'NONE', #16136, 8.300000000000000711 ) ;
#147649=CIRCLE ( 'NONE', #158011, 6.399999999999999467 ) ;
#147733=ORIENTED_EDGE ( 'NONE', *, *, #11410, .T. ) ;
#147855=EDGE_CURVE ( 'NONE', #212637, #71815, #147649, .T. ) ;
#149083=ORIENTED_EDGE ( 'NONE', *, *, #181903, .F. ) ;
#149472=DIRECTION ( 'NONE',  ( 0.000000000000000000, 0.000000000000000000, 1.000000000000000000 ) ) ;
#149498=CARTESIAN_POINT ( 'NONE',  ( 0.000000000000000000, 10.00000000000000888, 0.000000000000000000 ) ) ;
#149611=VERTEX_POINT ( 'NONE', #158954 ) ;
#149612=ORIENTED_EDGE ( 'NONE', *, *, #80870, .T. ) ;
#150340=DIRECTION ( 'NONE',  ( -1.224646799147353207E-16, 0.000000000000000000, -1.000000000000000000 ) ) ;
#150501=LINE ( 'NONE', #83331, #145031 ) ;
#150552=FACE_OUTER_BOUND ( 'NONE', #123608, .T. ) ;
#150598=CIRCLE ( 'NONE', #8641, 4.500000000000000000 ) ;
#151075=CYLINDRICAL_SURFACE ( 'NONE', #159965, 8.500000000000000000 ) ;
#151279=COLOUR_RGB ( '', 0.72549020, 0.75294118, 0.79215686) ;
#151465=AXIS2_PLACEMENT_3D ( 'NONE', #127828, #30232, #78964 ) ;
#151668=ORIENTED_EDGE ( 'NONE', *, *, #2591, .T. ) ;
#151851=ORIENTED_EDGE ( 'NONE', *, *, #87756, .T. ) ;
#151982=PRESENTATION_STYLE_ASSIGNMENT (( #168224 ) ) ;
#152191=( GEOMETRIC_REPRESENTATION_CONTEXT ( 3 ) GLOBAL_UNCERTAINTY_ASSIGNED_CONTEXT ( ( #65544 ) ) GLOBAL_UNIT_ASSIGNED_CONTEXT ( ( #116330, #345, #50211 ) ) REPRESENTATION_CONTEXT ( 'NONE', 'WORKASPACE' ) );
#152690=DIRECTION ( 'NONE',  ( 0.000000000000000000, 0.000000000000000000, -1.000000000000000000 ) ) ;
#153001=ADVANCED_FACE ( 'NONE', ( #210173 ), #40809, .T. ) ;
#153041=DIRECTION ( 'NONE',  ( 0.000000000000000000, 0.000000000000000000, 1.000000000000000000 ) ) ;
#153201=AXIS2_PLACEMENT_3D ( 'NONE', #69541, #82609, #32807 ) ;
#154101=TOROIDAL_SURFACE ( 'NONE', #26067, 6.399999999999999467, 0.2000000000000000111 ) ;
#154845=CARTESIAN_POINT ( 'NONE',  ( 0.000000000000000000, -3.600000000000005862, -4.899999999999999467 ) ) ;
#155052=ORIENTED_EDGE ( 'NONE', *, *, #176811, .F. ) ;
#155330=VERTEX_POINT ( 'NONE', #76218 ) ;
#155824=ORIENTED_EDGE ( 'NONE', *, *, #200474, .T. ) ;
#156266=ORIENTED_EDGE ( 'NONE', *, *, #188595, .F. ) ;
#156390=FACE_OUTER_BOUND ( 'NONE', #62703, .T. ) ;
#157520=EDGE_CURVE ( 'NONE', #83982, #185214, #91569, .T. ) ;
#158011=AXIS2_PLACEMENT_3D ( 'NONE', #56102, #203383, #186083 ) ;
#158265=DIRECTION ( 'NONE',  ( 0.000000000000000000, -1.000000000000000000, 0.000000000000000000 ) ) ;
#158440=DIRECTION ( 'NONE',  ( 0.000000000000000000, 0.000000000000000000, 1.000000000000000000 ) ) ;
#158513=EDGE_LOOP ( 'NONE', ( #122636, #200847 ) ) ;
#158954=CARTESIAN_POINT ( 'NONE',  ( 1.040949779275250140E-15, 0.2000000000000057288, 8.500000000000000000 ) ) ;
#159598=ORIENTED_EDGE ( 'NONE', *, *, #574, .F. ) ;
#159621=CARTESIAN_POINT ( 'NONE',  ( 0.000000000000000000, -4.000000000000003553, 0.000000000000000000 ) ) ;
#159965=AXIS2_PLACEMENT_3D ( 'NONE', #19971, #36222, #118618 ) ;
#160121=CARTESIAN_POINT ( 'NONE',  ( 0.000000000000000000, -4.000000000000003553, 0.000000000000000000 ) ) ;
#160473=DIRECTION ( 'NONE',  ( 1.224646799147353207E-16, 0.000000000000000000, -1.000000000000000000 ) ) ;
#160788=ORIENTED_EDGE ( 'NONE', *, *, #162297, .T. ) ;
#161266=DIRECTION ( 'NONE',  ( 1.000000000000000000, 0.000000000000000000, 0.000000000000000000 ) ) ;
#161654=MECHANICAL_DESIGN_GEOMETRIC_PRESENTATION_REPRESENTATION('',(#71617),#5884);
#162297=EDGE_CURVE ( 'NONE', #83982, #8134, #97143, .T. ) ;
#162306=CARTESIAN_POINT ( 'NONE',  ( 0.000000000000000000, 7.999999999999992895, 0.000000000000000000 ) ) ;
#162520=CARTESIAN_POINT ( 'NONE',  ( 0.000000000000000000, -0.2000000000000057288, 6.200000000000000178 ) ) ;
#162661=DIRECTION ( 'NONE',  ( 0.000000000000000000, 0.000000000000000000, 1.000000000000000000 ) ) ;
#162697=DIRECTION ( 'NONE',  ( 0.000000000000000000, -1.000000000000000000, 0.000000000000000000 ) ) ;
#162745=DIRECTION ( 'NONE',  ( 0.000000000000000000, 0.000000000000000000, -1.000000000000000000 ) ) ;
#163561=EDGE_CURVE ( 'NONE', #130319, #149611, #135162, .T. ) ;
#163746=VERTEX_POINT ( 'NONE', #178355 ) ;
#163853=CYLINDRICAL_SURFACE ( 'NONE', #25000, 4.500000000000000000 ) ;
#163856=DIRECTION ( 'NONE',  ( 0.000000000000000000, 1.000000000000000000, 0.000000000000000000 ) ) ;
#164446=AXIS2_PLACEMENT_3D ( 'NONE', #110701, #195083, #29391 ) ;
#164766=ADVANCED_FACE ( 'NONE', ( #81525 ), #130356, .T. ) ;
#164855=VERTEX_POINT ( 'NONE', #16497 ) ;
#165204=UNCERTAINTY_MEASURE_WITH_UNIT (LENGTH_MEASURE( 1.000000000000000082E-05 ), #49154, 'distance_accuracy_value', 'NONE');
#166470=TOROIDAL_SURFACE ( 'NONE', #7360, 7.750000000000000888, 0.7500000000000000000 ) ;
#166851=CARTESIAN_POINT ( 'NONE',  ( 0.000000000000000000, 7.999999999999992895, 0.000000000000000000 ) ) ;
#167164=( NAMED_UNIT ( * ) PLANE_ANGLE_UNIT ( ) SI_UNIT ( $, .RADIAN. ) );
#168224=SURFACE_STYLE_USAGE ( .BOTH. , #102157 ) ;
#168926=ORIENTED_EDGE ( 'NONE', *, *, #16828, .F. ) ;
#169271=CARTESIAN_POINT ( 'NONE',  ( 0.000000000000000000, -4.000000000000003553, -5.799999999999999822 ) ) ;
#169299=CARTESIAN_POINT ( 'NONE',  ( 0.000000000000000000, 7.999999999999992895, -8.500000000000000000 ) ) ;
#169504=ORIENTED_EDGE ( 'NONE', *, *, #192353, .F. ) ;
#169602=APPLICATION_CONTEXT ( 'automotive_design' ) ;
#170558=AXIS2_PLACEMENT_3D ( 'NONE', #38330, #34059, #53512 ) ;
#170575=EDGE_CURVE ( 'NONE', #26370, #155330, #14188, .T. ) ;
#171249=CIRCLE ( 'NONE', #101992, 7.750000000000000888 ) ;
#171269=LINE ( 'NONE', #25013, #34430 ) ;
#171652=ADVANCED_FACE ( 'NONE', ( #156390 ), #190991, .T. ) ;
#172394=DIRECTION ( 'NONE',  ( 0.000000000000000000, 0.000000000000000000, 1.000000000000000000 ) ) ;
#172561=DIRECTION ( 'NONE',  ( 0.000000000000000000, 1.000000000000000000, 0.000000000000000000 ) ) ;
#172991=VERTEX_POINT ( 'NONE', #169271 ) ;
#173170=CARTESIAN_POINT ( 'NONE',  ( 9.491012693391987787E-16, 7.250000000000006217, -7.750000000000000888 ) ) ;
#173536=EDGE_LOOP ( 'NONE', ( #178853, #135172, #205470, #39310 ) ) ;
#174308=TOROIDAL_SURFACE ( 'NONE', #25539, 8.300000000000000711, 0.2000000000000000111 ) ;
#174578=CIRCLE ( 'NONE', #18967, 4.899999999999999467 ) ;
#175177=ORIENTED_EDGE ( 'NONE', *, *, #179502, .F. ) ;
#175392=DIRECTION ( 'NONE',  ( 1.000000000000000000, -0.000000000000000000, 1.224646799147353207E-16 ) ) ;
#175406=EDGE_CURVE ( 'NONE', #140029, #132973, #125470, .T. ) ;
#175570=ORIENTED_EDGE ( 'NONE', *, *, #188595, .T. ) ;
#175767=CARTESIAN_POINT ( 'NONE',  ( 0.000000000000000000, -0.2000000000000057288, 0.000000000000000000 ) ) ;
#176127=AXIS2_PLACEMENT_3D ( 'NONE', #191951, #162697, #59841 ) ;
#176228=CIRCLE ( 'NONE', #203858, 5.799999999999999822 ) ;
#176527=ORIENTED_EDGE ( 'NONE', *, *, #157520, .T. ) ;
#176786=ORIENTED_EDGE ( 'NONE', *, *, #188776, .F. ) ;
#176811=EDGE_CURVE ( 'NONE', #185214, #20648, #25180, .T. ) ;
#176945=EDGE_CURVE ( 'NONE', #163746, #72143, #53318, .T. ) ;
#177071=ORIENTED_EDGE ( 'NONE', *, *, #130371, .T. ) ;
#177396=CONICAL_SURFACE ( 'NONE', #45996, 4.500000000000000000, 0.7853981633974491672 ) ;
#177846=ORIENTED_EDGE ( 'NONE', *, *, #63620, .F. ) ;
#177931=ORIENTED_EDGE ( 'NONE', *, *, #197101, .T. ) ;
#178313=DIRECTION ( 'NONE',  ( -0.000000000000000000, -1.000000000000000000, -0.000000000000000000 ) ) ;
#178355=CARTESIAN_POINT ( 'NONE',  ( 5.510910596163088569E-16, 6.999999999999992006, 4.500000000000000000 ) ) ;
#178622=CARTESIAN_POINT ( 'NONE',  ( 0.000000000000000000, 7.250000000000006217, 0.000000000000000000 ) ) ;
#178853=ORIENTED_EDGE ( 'NONE', *, *, #65319, .F. ) ;
#178931=PLANE ( 'NONE',  #15171 ) ;
#179502=EDGE_CURVE ( 'NONE', #140029, #149611, #195153, .T. ) ;
#179626=EDGE_CURVE ( 'NONE', #80292, #130319, #70299, .T. ) ;
#180269=CARTESIAN_POINT ( 'NONE',  ( 0.000000000000000000, 0.2000000000000057288, -8.500000000000000000 ) ) ;
#180474=SURFACE_STYLE_USAGE ( .BOTH. , #114475 ) ;
#180628=ORIENTED_EDGE ( 'NONE', *, *, #200627, .F. ) ;
#180798=DIRECTION ( 'NONE',  ( -0.000000000000000000, -1.000000000000000000, -0.000000000000000000 ) ) ;
#181091=TOROIDAL_SURFACE ( 'NONE', #170558, 5.799999999999999822, 0.4000000000000000222 ) ;
#181551=AXIS2_PLACEMENT_3D ( 'NONE', #14011, #180798, #32423 ) ;
#181903=EDGE_CURVE ( 'NONE', #212637, #93781, #111978, .T. ) ;
#182300=EDGE_CURVE ( 'NONE', #186457, #172991, #63508, .T. ) ;
#182755=DIRECTION ( 'NONE',  ( 0.000000000000000000, 1.000000000000000000, 0.000000000000000000 ) ) ;
#182770=DIRECTION ( 'NONE',  ( -0.000000000000000000, -1.000000000000000000, -0.000000000000000000 ) ) ;
#183309=DIRECTION ( 'NONE',  ( 0.000000000000000000, 0.7071067811865469066, 0.7071067811865481278 ) ) ;
#185205=FACE_OUTER_BOUND ( 'NONE', #158513, .T. ) ;
#185214=VERTEX_POINT ( 'NONE', #190161 ) ;
#185472=ORIENTED_EDGE ( 'NONE', *, *, #10274, .T. ) ;
#185842=DIRECTION ( 'NONE',  ( 0.000000000000000000, 1.000000000000000000, 0.000000000000000000 ) ) ;
#185906=CIRCLE ( 'NONE', #92573, 5.799999999999999822 ) ;
#186083=DIRECTION ( 'NONE',  ( 0.000000000000000000, 0.000000000000000000, 1.000000000000000000 ) ) ;
#186216=CARTESIAN_POINT ( 'NONE',  ( 0.000000000000000000, -3.600000000000005862, 0.000000000000000000 ) ) ;
#186254=DIRECTION ( 'NONE',  ( 0.000000000000000000, 0.000000000000000000, 1.000000000000000000 ) ) ;
#186309=DIRECTION ( 'NONE',  ( -1.000000000000000000, 0.000000000000000000, 0.000000000000000000 ) ) ;
#186457=VERTEX_POINT ( 'NONE', #38119 ) ;
#187447=ADVANCED_FACE ( 'NONE', ( #66252 ), #70727, .T. ) ;
#187797=DIRECTION ( 'NONE',  ( 0.000000000000000000, 1.000000000000000000, 0.000000000000000000 ) ) ;
#188047=AXIS2_PLACEMENT_3D ( 'NONE', #202577, #20632, #109188 ) ;
#188305=SHAPE_REPRESENTATION ( 'drip tip', ( #200407 ), #152191 ) ;
#188407=AXIS2_PLACEMENT_3D ( 'NONE', #147364, #213390, #15196 ) ;
#188449=CARTESIAN_POINT ( 'NONE',  ( 0.000000000000000000, 0.2000000000000057288, 0.000000000000000000 ) ) ;
#188585=DIRECTION ( 'NONE',  ( 0.000000000000000000, 1.000000000000000000, 0.000000000000000000 ) ) ;
#188595=EDGE_CURVE ( 'NONE', #140029, #127623, #39682, .T. ) ;
#188776=EDGE_CURVE ( 'NONE', #126977, #149611, #53589, .T. ) ;
#188799=DIRECTION ( 'NONE',  ( 0.000000000000000000, 0.000000000000000000, -1.000000000000000000 ) ) ;
#189062=CARTESIAN_POINT ( 'NONE',  ( 0.000000000000000000, 7.999999999999992895, 0.000000000000000000 ) ) ;
#189849=ADVANCED_FACE ( 'NONE', ( #204591 ), #154101, .F. ) ;
#189939=DIRECTION ( 'NONE',  ( 0.000000000000000000, 0.000000000000000000, 1.000000000000000000 ) ) ;
#190161=CARTESIAN_POINT ( 'NONE',  ( 0.000000000000000000, -3.600000000000005862, -4.500000000000000000 ) ) ;
#190333=LINE ( 'NONE', #91812, #73702 ) ;
#190373=COLOUR_RGB ( '', 0.72549020, 0.75294118, 0.79215686) ;
#190991=CYLINDRICAL_SURFACE ( 'NONE', #17738, 6.200000000000000178 ) ;
#191106=DIRECTION ( 'NONE',  ( 0.000000000000000000, 0.000000000000000000, 1.000000000000000000 ) ) ;
#191183=EDGE_CURVE ( 'NONE', #26370, #186457, #133415, .T. ) ;
#191810=AXIS2_PLACEMENT_3D ( 'NONE', #2320, #82529, #162745 ) ;
#191922=CARTESIAN_POINT ( 'NONE',  ( 1.040949779275250140E-15, 7.999999999999992895, 8.500000000000000000 ) ) ;
#191951=CARTESIAN_POINT ( 'NONE',  ( 0.000000000000000000, 7.999999999999992895, 0.000000000000000000 ) ) ;
#192040=CARTESIAN_POINT ( 'NONE',  ( 0.000000000000000000, 0.000000000000000000, 0.000000000000000000 ) ) ;
#192353=EDGE_CURVE ( 'NONE', #127623, #126977, #100037, .T. ) ;
#192403=ORIENTED_EDGE ( 'NONE', *, *, #176945, .F. ) ;
#193078=AXIS2_PLACEMENT_3D ( 'NONE', #92213, #158265, #9854 ) ;
#193130=CARTESIAN_POINT ( 'NONE',  ( 0.000000000000000000, 7.999999999999992895, 7.750000000000000888 ) ) ;
#193179=DIRECTION ( 'NONE',  ( -0.000000000000000000, 1.000000000000000000, -0.000000000000000000 ) ) ;
#193722=DIRECTION ( 'NONE',  ( 0.000000000000000000, 1.000000000000000000, 0.000000000000000000 ) ) ;
#194160=TOROIDAL_SURFACE ( 'NONE', #114745, 6.399999999999999467, 0.2000000000000000111 ) ;
#194198=DIRECTION ( 'NONE',  ( 0.000000000000000000, 0.000000000000000000, -1.000000000000000000 ) ) ;
#194629=AXIS2_PLACEMENT_3D ( 'NONE', #48862, #14192, #160473 ) ;
#195083=DIRECTION ( 'NONE',  ( -0.000000000000000000, 1.000000000000000000, -0.000000000000000000 ) ) ;
#195153=LINE ( 'NONE', #191922, #8001 ) ;
#195307=ORIENTED_EDGE ( 'NONE', *, *, #23415, .F. ) ;
#195967=CIRCLE ( 'NONE', #119946, 6.399999999999999467 ) ;
#196348=CARTESIAN_POINT ( 'NONE',  ( 0.000000000000000000, -4.000000000000003553, 0.000000000000000000 ) ) ;
#197101=EDGE_CURVE ( 'NONE', #130319, #80292, #147611, .T. ) ;
#197146=ADVANCED_FACE ( 'NONE', ( #150552 ), #133861, .T. ) ;
#197608=DIRECTION ( 'NONE',  ( 0.000000000000000000, 0.000000000000000000, 1.000000000000000000 ) ) ;
#198166=AXIS2_PLACEMENT_3D ( 'NONE', #100775, #136499, #17374 ) ;
#199358=AXIS2_PLACEMENT_3D ( 'NONE', #7671, #139851, #141998 ) ;
#199633=FILL_AREA_STYLE ('',( #53399 ) ) ;
#199703=CARTESIAN_POINT ( 'NONE',  ( 0.000000000000000000, -3.600000000000005862, 0.000000000000000000 ) ) ;
#200066=DIRECTION ( 'NONE',  ( 0.000000000000000000, 0.000000000000000000, 1.000000000000000000 ) ) ;
#200201=VERTEX_POINT ( 'NONE', #86301 ) ;
#200207=CIRCLE ( 'NONE', #41149, 6.200000000000000178 ) ;
#200386=PLANE ( 'NONE',  #45992 ) ;
#200407=AXIS2_PLACEMENT_3D ( 'NONE', #95216, #132002, #161266 ) ;
#200474=EDGE_CURVE ( 'NONE', #155330, #172991, #185906, .T. ) ;
#200524=CARTESIAN_POINT ( 'NONE',  ( 0.000000000000000000, -0.2000000000000057288, 0.000000000000000000 ) ) ;
#200627=EDGE_CURVE ( 'NONE', #163746, #23490, #89166, .T. ) ;
#200761=DIRECTION ( 'NONE',  ( -0.000000000000000000, 1.000000000000000000, -0.000000000000000000 ) ) ;
#200847=ORIENTED_EDGE ( 'NONE', *, *, #119697, .T. ) ;
#201209=APPLICATION_CONTEXT ( 'automotive_design' ) ;
#201906=ORIENTED_EDGE ( 'NONE', *, *, #176811, .T. ) ;
#202164=ORIENTED_EDGE ( 'NONE', *, *, #91398, .T. ) ;
#202577=CARTESIAN_POINT ( 'NONE',  ( 0.000000000000000000, 0.2000000000000057288, 0.000000000000000000 ) ) ;
#203281=EDGE_LOOP ( 'NONE', ( #101870, #177071, #145248, #79202 ) ) ;
#203383=DIRECTION ( 'NONE',  ( 0.000000000000000000, 1.000000000000000000, 0.000000000000000000 ) ) ;
#203858=AXIS2_PLACEMENT_3D ( 'NONE', #121754, #89189, #188799 ) ;
#203951=CARTESIAN_POINT ( 'NONE',  ( 0.000000000000000000, 6.999999999999992006, -4.500000000000000000 ) ) ;
#204591=FACE_OUTER_BOUND ( 'NONE', #210625, .T. ) ;
#205318=LINE ( 'NONE', #75338, #7758 ) ;
#205470=ORIENTED_EDGE ( 'NONE', *, *, #181903, .T. ) ;
#205761=CARTESIAN_POINT ( 'NONE',  ( 0.000000000000000000, 7.250000000000006217, 7.750000000000000888 ) ) ;
#207931=CARTESIAN_POINT ( 'NONE',  ( 6.000769315822030740E-16, -4.000000000000005329, 4.899999999999999467 ) ) ;
#207947=ORIENTED_EDGE ( 'NONE', *, *, #1373, .T. ) ;
#208584=ORIENTED_EDGE ( 'NONE', *, *, #200627, .T. ) ;
#209645=ORIENTED_EDGE ( 'NONE', *, *, #191183, .T. ) ;
#210018=FACE_OUTER_BOUND ( 'NONE', #83645, .T. ) ;
#210173=FACE_OUTER_BOUND ( 'NONE', #140975, .T. ) ;
#210209=EDGE_LOOP ( 'NONE', ( #151668, #126378, #207947, #169504 ) ) ;
#210625=EDGE_LOOP ( 'NONE', ( #168926, #110009, #46679, #149083 ) ) ;
#211433=EDGE_LOOP ( 'NONE', ( #105980, #28786, #131803, #176786 ) ) ;
#212026=EDGE_LOOP ( 'NONE', ( #16964, #26099 ) ) ;
#212637=VERTEX_POINT ( 'NONE', #8319 ) ;
#213390=DIRECTION ( 'NONE',  ( 0.000000000000000000, 1.000000000000000000, 0.000000000000000000 ) ) ;
ENDSEC;
END-ISO-10303-21;
